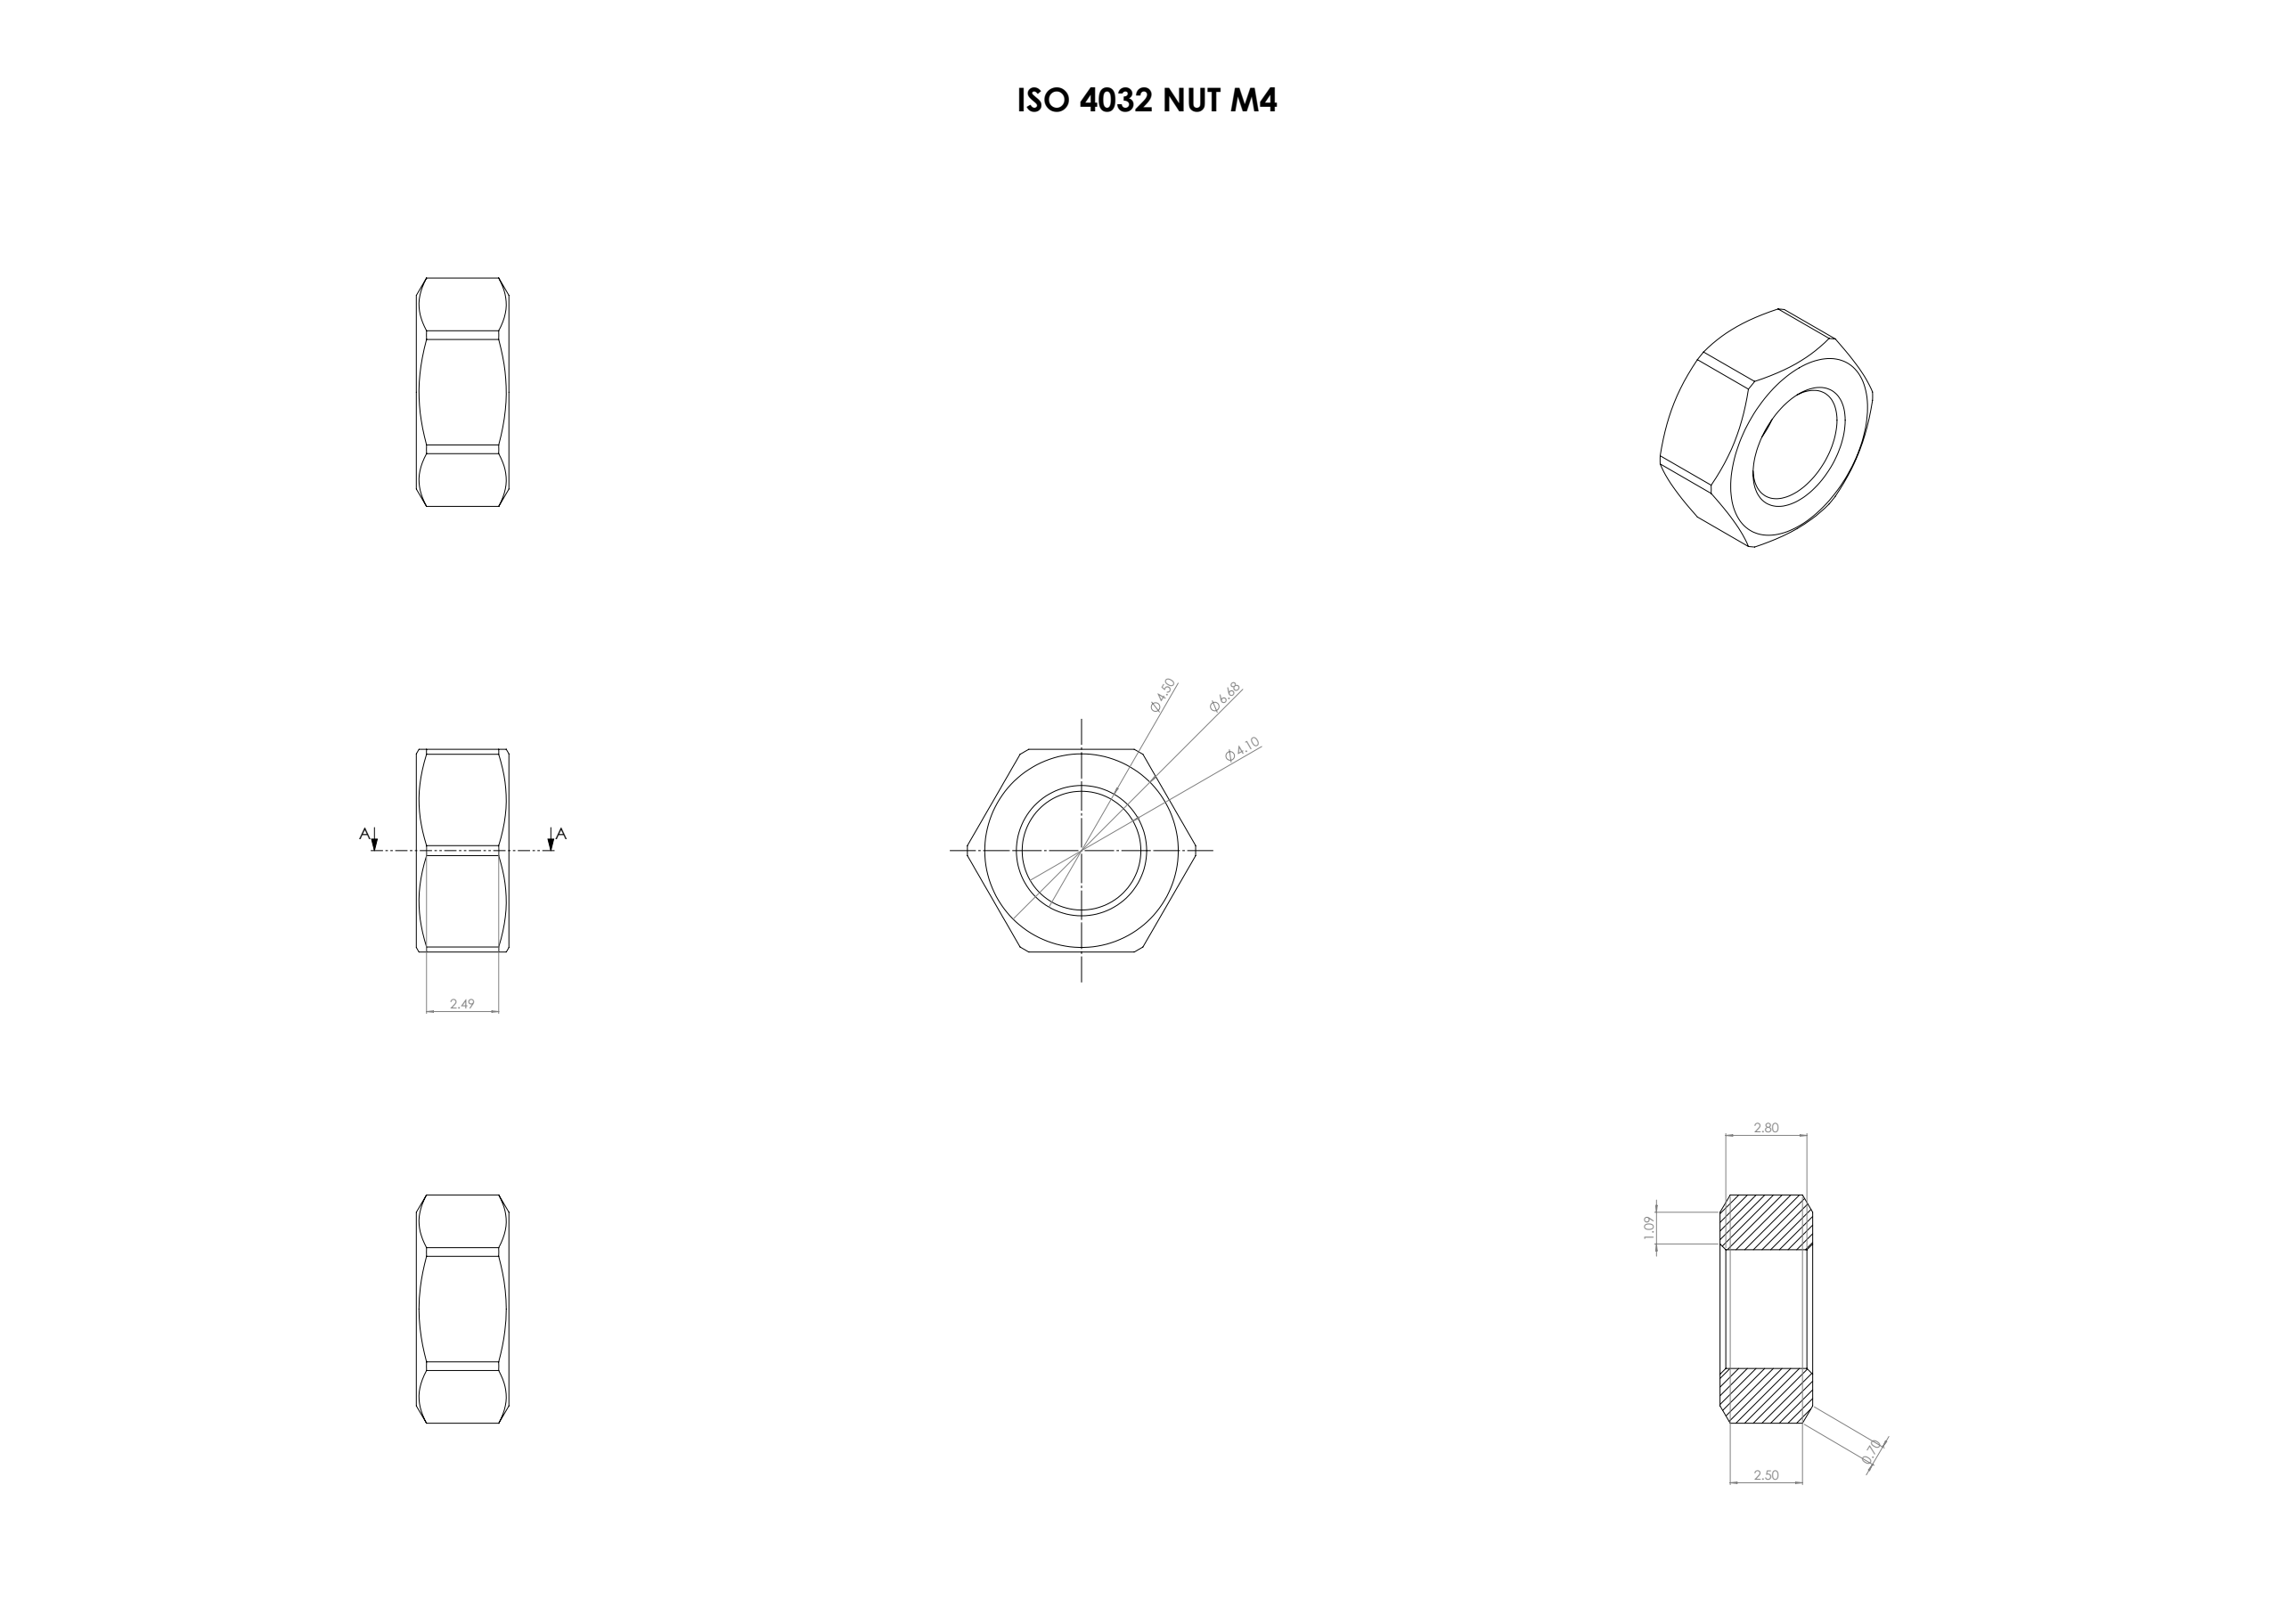
ISO-10303-21;
HEADER;
/* Generated by software containing ST-Developer
 * from STEP Tools, Inc. (www.steptools.com) 
 */

FILE_DESCRIPTION(
/* description */ (''),
/* implementation_level */ '2;1');

FILE_NAME(
/* name */ '10_ISO_4032_Nut_M4.step',
/* time_stamp */ '2026-10-21T02:01:14-07:00',
/* author */ (''),
/* organization */ (''),
/* preprocessor_version */ 'ST-DEVELOPER v20.2',
/* originating_system */ 'Autodesk Translation Framework v15.15.0.0',
/* authorisation */ '');

FILE_SCHEMA (('AUTOMOTIVE_DESIGN { 1 0 10303 214 3 1 1 }'));
ENDSEC;

DATA;
#10=MECHANICAL_DESIGN_GEOMETRIC_PRESENTATION_REPRESENTATION('',(#625),#37181);
#599=SHAPE_REPRESENTATION_RELATIONSHIP('SRR','None',#37249,#612);
#612=ADVANCED_BREP_SHAPE_REPRESENTATION('',(#638),#37179);
#625=STYLED_ITEM('',(#37380),#638);
#638=MANIFOLD_SOLID_BREP('Body1',#14787);
#686=FACE_BOUND('',#3028,.T.);
#687=FACE_BOUND('',#3031,.T.);
#912=CYLINDRICAL_SURFACE('',#16021,2.05);
#1265=CIRCLE('',#16017,3.34203030879952);
#1266=CIRCLE('',#16019,2.25);
#1267=CIRCLE('',#16020,2.05);
#1268=CIRCLE('',#16022,2.05);
#1269=CIRCLE('',#16024,3.34203030879952);
#1270=CIRCLE('',#16026,2.25);
#1362=CONICAL_SURFACE('',#16016,3.83322594216369,1.03985037524359);
#1363=CONICAL_SURFACE('',#16018,2.15,0.785398163397448);
#1364=CONICAL_SURFACE('',#16025,2.15,0.785398163397448);
#1365=CONICAL_SURFACE('',#16030,3.83322594216369,1.03985037524359);
#2136=FACE_OUTER_BOUND('',#3022,.T.);
#2137=FACE_OUTER_BOUND('',#3023,.T.);
#2138=FACE_OUTER_BOUND('',#3024,.T.);
#2139=FACE_OUTER_BOUND('',#3025,.T.);
#2140=FACE_OUTER_BOUND('',#3026,.T.);
#2141=FACE_OUTER_BOUND('',#3027,.T.);
#2142=FACE_OUTER_BOUND('',#3029,.T.);
#2143=FACE_OUTER_BOUND('',#3030,.T.);
#2144=FACE_OUTER_BOUND('',#3032,.T.);
#2145=FACE_OUTER_BOUND('',#3033,.T.);
#2146=FACE_OUTER_BOUND('',#3034,.T.);
#2147=FACE_OUTER_BOUND('',#3035,.T.);
#2148=FACE_OUTER_BOUND('',#3036,.T.);
#2149=FACE_OUTER_BOUND('',#3037,.T.);
#2150=FACE_OUTER_BOUND('',#3038,.T.);
#2151=FACE_OUTER_BOUND('',#3039,.T.);
#2152=FACE_OUTER_BOUND('',#3040,.T.);
#2153=FACE_OUTER_BOUND('',#3041,.T.);
#2154=FACE_OUTER_BOUND('',#3042,.T.);
#3022=EDGE_LOOP('',(#13069,#13070,#13071,#13072));
#3023=EDGE_LOOP('',(#13073,#13074,#13075,#13076));
#3024=EDGE_LOOP('',(#13077,#13078,#13079,#13080,#13081,#13082,#13083,#13084,
#13085,#13086,#13087,#13088,#13089,#13090,#13091,#13092));
#3025=EDGE_LOOP('',(#13093,#13094,#13095,#13096));
#3026=EDGE_LOOP('',(#13097,#13098,#13099,#13100));
#3027=EDGE_LOOP('',(#13101));
#3028=EDGE_LOOP('',(#13102));
#3029=EDGE_LOOP('',(#13103,#13104,#13105,#13106));
#3030=EDGE_LOOP('',(#13107));
#3031=EDGE_LOOP('',(#13108));
#3032=EDGE_LOOP('',(#13109,#13110,#13111,#13112));
#3033=EDGE_LOOP('',(#13113,#13114,#13115,#13116));
#3034=EDGE_LOOP('',(#13117,#13118,#13119,#13120,#13121,#13122,#13123,#13124,
#13125,#13126,#13127,#13128,#13129,#13130,#13131,#13132));
#3035=EDGE_LOOP('',(#13133,#13134,#13135,#13136));
#3036=EDGE_LOOP('',(#13137,#13138,#13139,#13140,#13141,#13142));
#3037=EDGE_LOOP('',(#13143,#13144,#13145,#13146));
#3038=EDGE_LOOP('',(#13147,#13148,#13149,#13150));
#3039=EDGE_LOOP('',(#13151,#13152,#13153,#13154));
#3040=EDGE_LOOP('',(#13155,#13156,#13157,#13158));
#3041=EDGE_LOOP('',(#13159,#13160,#13161,#13162));
#3042=EDGE_LOOP('',(#13163,#13164,#13165,#13166));
#3176=(
BOUNDED_CURVE()
B_SPLINE_CURVE(2,(#34308,#34309,#34310),.UNSPECIFIED.,.F.,.F.)
B_SPLINE_CURVE_WITH_KNOTS((3,3),(0.0719702485074244,0.107109429758004),
 .UNSPECIFIED.)
CURVE()
GEOMETRIC_REPRESENTATION_ITEM()
RATIONAL_B_SPLINE_CURVE((1.0121972483025,1.01317411304727,1.0121972483025))
REPRESENTATION_ITEM('')
);
#3177=(
BOUNDED_CURVE()
B_SPLINE_CURVE(2,(#34314,#34315,#34316),.UNSPECIFIED.,.F.,.F.)
B_SPLINE_CURVE_WITH_KNOTS((3,3),(0.0719702485074238,0.107109429758003),
 .UNSPECIFIED.)
CURVE()
GEOMETRIC_REPRESENTATION_ITEM()
RATIONAL_B_SPLINE_CURVE((1.0121972483025,1.01317411304726,1.0121972483025))
REPRESENTATION_ITEM('')
);
#3178=(
BOUNDED_CURVE()
B_SPLINE_CURVE(2,(#34320,#34321,#34322),.UNSPECIFIED.,.F.,.F.)
B_SPLINE_CURVE_WITH_KNOTS((3,3),(0.0663017168058462,0.456855245466122),
 .UNSPECIFIED.)
CURVE()
GEOMETRIC_REPRESENTATION_ITEM()
RATIONAL_B_SPLINE_CURVE((1.05321457643448,1.18720024765905,1.05321457643448))
REPRESENTATION_ITEM('')
);
#3179=(
BOUNDED_CURVE()
B_SPLINE_CURVE(2,(#34325,#34326,#34327),.UNSPECIFIED.,.F.,.F.)
B_SPLINE_CURVE_WITH_KNOTS((3,3),(0.0663017168058461,0.456855245466121),
 .UNSPECIFIED.)
CURVE()
GEOMETRIC_REPRESENTATION_ITEM()
RATIONAL_B_SPLINE_CURVE((1.05321457643448,1.18720024765905,1.05321457643448))
REPRESENTATION_ITEM('')
);
#3180=(
BOUNDED_CURVE()
B_SPLINE_CURVE(2,(#34330,#34331,#34332),.UNSPECIFIED.,.F.,.F.)
B_SPLINE_CURVE_WITH_KNOTS((3,3),(0.0663017168058462,0.456855245466121),
 .UNSPECIFIED.)
CURVE()
GEOMETRIC_REPRESENTATION_ITEM()
RATIONAL_B_SPLINE_CURVE((1.05321457643448,1.18720024765905,1.05321457643448))
REPRESENTATION_ITEM('')
);
#3181=(
BOUNDED_CURVE()
B_SPLINE_CURVE(2,(#34334,#34335,#34336),.UNSPECIFIED.,.F.,.F.)
B_SPLINE_CURVE_WITH_KNOTS((3,3),(0.0719702485074243,0.107109429758004),
 .UNSPECIFIED.)
CURVE()
GEOMETRIC_REPRESENTATION_ITEM()
RATIONAL_B_SPLINE_CURVE((1.0121972483025,1.01317411304726,1.0121972483025))
REPRESENTATION_ITEM('')
);
#3182=(
BOUNDED_CURVE()
B_SPLINE_CURVE(2,(#34338,#34339,#34340),.UNSPECIFIED.,.F.,.F.)
B_SPLINE_CURVE_WITH_KNOTS((3,3),(0.0663017168058464,0.456855245466122),
 .UNSPECIFIED.)
CURVE()
GEOMETRIC_REPRESENTATION_ITEM()
RATIONAL_B_SPLINE_CURVE((1.05321457643448,1.18720024765905,1.05321457643448))
REPRESENTATION_ITEM('')
);
#3183=(
BOUNDED_CURVE()
B_SPLINE_CURVE(2,(#34342,#34343,#34344),.UNSPECIFIED.,.F.,.F.)
B_SPLINE_CURVE_WITH_KNOTS((3,3),(0.0719702485074242,0.107109429758004),
 .UNSPECIFIED.)
CURVE()
GEOMETRIC_REPRESENTATION_ITEM()
RATIONAL_B_SPLINE_CURVE((1.0121972483025,1.01317411304726,1.0121972483025))
REPRESENTATION_ITEM('')
);
#3184=(
BOUNDED_CURVE()
B_SPLINE_CURVE(2,(#34346,#34347,#34348),.UNSPECIFIED.,.F.,.F.)
B_SPLINE_CURVE_WITH_KNOTS((3,3),(0.261578481135983,0.456855245466121),
 .UNSPECIFIED.)
CURVE()
GEOMETRIC_REPRESENTATION_ITEM()
RATIONAL_B_SPLINE_CURVE((1.12020741204677,1.12020741204677,1.05321457643449))
REPRESENTATION_ITEM('')
);
#3185=(
BOUNDED_CURVE()
B_SPLINE_CURVE(2,(#34353,#34354,#34355),.UNSPECIFIED.,.F.,.F.)
B_SPLINE_CURVE_WITH_KNOTS((3,3),(0.0663017168058461,0.261578481135983),
 .UNSPECIFIED.)
CURVE()
GEOMETRIC_REPRESENTATION_ITEM()
RATIONAL_B_SPLINE_CURVE((1.05321457643448,1.12020741204677,1.12020741204677))
REPRESENTATION_ITEM('')
);
#3186=(
BOUNDED_CURVE()
B_SPLINE_CURVE(2,(#34357,#34358,#34359),.UNSPECIFIED.,.F.,.F.)
B_SPLINE_CURVE_WITH_KNOTS((3,3),(0.0719702485074242,0.107109429758004),
 .UNSPECIFIED.)
CURVE()
GEOMETRIC_REPRESENTATION_ITEM()
RATIONAL_B_SPLINE_CURVE((1.0121972483025,1.01317411304727,1.0121972483025))
REPRESENTATION_ITEM('')
);
#3187=(
BOUNDED_CURVE()
B_SPLINE_CURVE(2,(#34361,#34362,#34363),.UNSPECIFIED.,.F.,.F.)
B_SPLINE_CURVE_WITH_KNOTS((3,3),(0.066301716805846,0.456855245466121),
 .UNSPECIFIED.)
CURVE()
GEOMETRIC_REPRESENTATION_ITEM()
RATIONAL_B_SPLINE_CURVE((1.05321457643448,1.18720024765905,1.05321457643448))
REPRESENTATION_ITEM('')
);
#3188=(
BOUNDED_CURVE()
B_SPLINE_CURVE(2,(#34365,#34366,#34367),.UNSPECIFIED.,.F.,.F.)
B_SPLINE_CURVE_WITH_KNOTS((3,3),(0.0719702485074249,0.107109429758004),
 .UNSPECIFIED.)
CURVE()
GEOMETRIC_REPRESENTATION_ITEM()
RATIONAL_B_SPLINE_CURVE((1.0121972483025,1.01317411304726,1.0121972483025))
REPRESENTATION_ITEM('')
);
#3189=(
BOUNDED_CURVE()
B_SPLINE_CURVE(2,(#34369,#34370,#34371),.UNSPECIFIED.,.F.,.F.)
B_SPLINE_CURVE_WITH_KNOTS((3,3),(0.0663017168058463,0.456855245466121),
 .UNSPECIFIED.)
CURVE()
GEOMETRIC_REPRESENTATION_ITEM()
RATIONAL_B_SPLINE_CURVE((1.05321457643448,1.18720024765905,1.05321457643448))
REPRESENTATION_ITEM('')
);
#3190=(
BOUNDED_CURVE()
B_SPLINE_CURVE(2,(#34372,#34373,#34374),.UNSPECIFIED.,.F.,.F.)
B_SPLINE_CURVE_WITH_KNOTS((3,3),(0.0719702485074235,0.107109429758003),
 .UNSPECIFIED.)
CURVE()
GEOMETRIC_REPRESENTATION_ITEM()
RATIONAL_B_SPLINE_CURVE((1.0121972483025,1.01317411304727,1.0121972483025))
REPRESENTATION_ITEM('')
);
#3191=(
BOUNDED_CURVE()
B_SPLINE_CURVE(2,(#34397,#34398,#34399),.UNSPECIFIED.,.F.,.F.)
B_SPLINE_CURVE_WITH_KNOTS((3,3),(0.0719702485074245,0.107109429758004),
 .UNSPECIFIED.)
CURVE()
GEOMETRIC_REPRESENTATION_ITEM()
RATIONAL_B_SPLINE_CURVE((1.0121972483025,1.01317411304727,1.0121972483025))
REPRESENTATION_ITEM('')
);
#3192=(
BOUNDED_CURVE()
B_SPLINE_CURVE(2,(#34403,#34404,#34405),.UNSPECIFIED.,.F.,.F.)
B_SPLINE_CURVE_WITH_KNOTS((3,3),(0.0663017168058461,0.456855245466121),
 .UNSPECIFIED.)
CURVE()
GEOMETRIC_REPRESENTATION_ITEM()
RATIONAL_B_SPLINE_CURVE((1.05321457643448,1.18720024765905,1.05321457643448))
REPRESENTATION_ITEM('')
);
#3193=(
BOUNDED_CURVE()
B_SPLINE_CURVE(2,(#34411,#34412,#34413),.UNSPECIFIED.,.F.,.F.)
B_SPLINE_CURVE_WITH_KNOTS((3,3),(0.0663017168058461,0.261578481135983),
 .UNSPECIFIED.)
CURVE()
GEOMETRIC_REPRESENTATION_ITEM()
RATIONAL_B_SPLINE_CURVE((1.05321457643448,1.12020741204677,1.12020741204677))
REPRESENTATION_ITEM('')
);
#3194=(
BOUNDED_CURVE()
B_SPLINE_CURVE(2,(#34414,#34415,#34416),.UNSPECIFIED.,.F.,.F.)
B_SPLINE_CURVE_WITH_KNOTS((3,3),(0.0719702485074254,0.107109429758005),
 .UNSPECIFIED.)
CURVE()
GEOMETRIC_REPRESENTATION_ITEM()
RATIONAL_B_SPLINE_CURVE((1.0121972483025,1.01317411304726,1.0121972483025))
REPRESENTATION_ITEM('')
);
#3195=(
BOUNDED_CURVE()
B_SPLINE_CURVE(2,(#34417,#34418,#34419),.UNSPECIFIED.,.F.,.F.)
B_SPLINE_CURVE_WITH_KNOTS((3,3),(0.0663017168058463,0.456855245466121),
 .UNSPECIFIED.)
CURVE()
GEOMETRIC_REPRESENTATION_ITEM()
RATIONAL_B_SPLINE_CURVE((1.05321457643448,1.18720024765905,1.05321457643448))
REPRESENTATION_ITEM('')
);
#3196=(
BOUNDED_CURVE()
B_SPLINE_CURVE(2,(#34421,#34422,#34423),.UNSPECIFIED.,.F.,.F.)
B_SPLINE_CURVE_WITH_KNOTS((3,3),(0.0719702485074251,0.107109429758005),
 .UNSPECIFIED.)
CURVE()
GEOMETRIC_REPRESENTATION_ITEM()
RATIONAL_B_SPLINE_CURVE((1.0121972483025,1.01317411304726,1.01219724830249))
REPRESENTATION_ITEM('')
);
#3197=(
BOUNDED_CURVE()
B_SPLINE_CURVE(2,(#34425,#34426,#34427),.UNSPECIFIED.,.F.,.F.)
B_SPLINE_CURVE_WITH_KNOTS((3,3),(0.0663017168058462,0.456855245466121),
 .UNSPECIFIED.)
CURVE()
GEOMETRIC_REPRESENTATION_ITEM()
RATIONAL_B_SPLINE_CURVE((1.05321457643448,1.18720024765905,1.05321457643448))
REPRESENTATION_ITEM('')
);
#3198=(
BOUNDED_CURVE()
B_SPLINE_CURVE(2,(#34429,#34430,#34431),.UNSPECIFIED.,.F.,.F.)
B_SPLINE_CURVE_WITH_KNOTS((3,3),(0.0719702485074238,0.107109429758004),
 .UNSPECIFIED.)
CURVE()
GEOMETRIC_REPRESENTATION_ITEM()
RATIONAL_B_SPLINE_CURVE((1.0121972483025,1.01317411304727,1.0121972483025))
REPRESENTATION_ITEM('')
);
#3199=(
BOUNDED_CURVE()
B_SPLINE_CURVE(2,(#34433,#34434,#34435),.UNSPECIFIED.,.F.,.F.)
B_SPLINE_CURVE_WITH_KNOTS((3,3),(0.0663017168058462,0.456855245466121),
 .UNSPECIFIED.)
CURVE()
GEOMETRIC_REPRESENTATION_ITEM()
RATIONAL_B_SPLINE_CURVE((1.05321457643448,1.18720024765905,1.05321457643448))
REPRESENTATION_ITEM('')
);
#3200=(
BOUNDED_CURVE()
B_SPLINE_CURVE(2,(#34437,#34438,#34439),.UNSPECIFIED.,.F.,.F.)
B_SPLINE_CURVE_WITH_KNOTS((3,3),(0.0719702485074251,0.107109429758005),
 .UNSPECIFIED.)
CURVE()
GEOMETRIC_REPRESENTATION_ITEM()
RATIONAL_B_SPLINE_CURVE((1.0121972483025,1.01317411304726,1.0121972483025))
REPRESENTATION_ITEM('')
);
#3201=(
BOUNDED_CURVE()
B_SPLINE_CURVE(2,(#34440,#34441,#34442),.UNSPECIFIED.,.F.,.F.)
B_SPLINE_CURVE_WITH_KNOTS((3,3),(0.261578481135983,0.456855245466121),
 .UNSPECIFIED.)
CURVE()
GEOMETRIC_REPRESENTATION_ITEM()
RATIONAL_B_SPLINE_CURVE((1.12020741204677,1.12020741204677,1.05321457643448))
REPRESENTATION_ITEM('')
);
#4375=LINE('',#34312,#5614);
#4376=LINE('',#34317,#5615);
#4377=LINE('',#34324,#5616);
#4378=LINE('',#34350,#5617);
#4379=LINE('',#34379,#5618);
#4380=LINE('',#34383,#5619);
#4381=LINE('',#34391,#5620);
#4382=LINE('',#34395,#5621);
#4383=LINE('',#34400,#5622);
#4384=LINE('',#34406,#5623);
#4385=LINE('',#34409,#5624);
#4386=LINE('',#34444,#5625);
#4387=LINE('',#34446,#5626);
#4388=LINE('',#34448,#5627);
#4389=LINE('',#34450,#5628);
#4390=LINE('',#34452,#5629);
#4391=LINE('',#34454,#5630);
#5614=VECTOR('',#19461,10.);
#5615=VECTOR('',#19462,10.);
#5616=VECTOR('',#19465,10.);
#5617=VECTOR('',#19468,3.83322594216369);
#5618=VECTOR('',#19475,2.15);
#5619=VECTOR('',#19480,2.05);
#5620=VECTOR('',#19491,2.15);
#5621=VECTOR('',#19496,10.);
#5622=VECTOR('',#19497,10.);
#5623=VECTOR('',#19500,10.);
#5624=VECTOR('',#19503,3.83322594216369);
#5625=VECTOR('',#19506,10.);
#5626=VECTOR('',#19509,10.);
#5627=VECTOR('',#19512,10.);
#5628=VECTOR('',#19515,10.);
#5629=VECTOR('',#19518,10.);
#5630=VECTOR('',#19521,10.);
#6898=VERTEX_POINT('',#34306);
#6899=VERTEX_POINT('',#34307);
#6900=VERTEX_POINT('',#34311);
#6901=VERTEX_POINT('',#34313);
#6902=VERTEX_POINT('',#34319);
#6903=VERTEX_POINT('',#34323);
#6904=VERTEX_POINT('',#34329);
#6905=VERTEX_POINT('',#34333);
#6906=VERTEX_POINT('',#34337);
#6907=VERTEX_POINT('',#34341);
#6908=VERTEX_POINT('',#34345);
#6909=VERTEX_POINT('',#34349);
#6910=VERTEX_POINT('',#34352);
#6911=VERTEX_POINT('',#34356);
#6912=VERTEX_POINT('',#34360);
#6913=VERTEX_POINT('',#34364);
#6914=VERTEX_POINT('',#34368);
#6915=VERTEX_POINT('',#34376);
#6916=VERTEX_POINT('',#34378);
#6917=VERTEX_POINT('',#34382);
#6918=VERTEX_POINT('',#34386);
#6919=VERTEX_POINT('',#34389);
#6920=VERTEX_POINT('',#34394);
#6921=VERTEX_POINT('',#34396);
#6922=VERTEX_POINT('',#34402);
#6923=VERTEX_POINT('',#34408);
#6924=VERTEX_POINT('',#34410);
#6925=VERTEX_POINT('',#34420);
#6926=VERTEX_POINT('',#34424);
#6927=VERTEX_POINT('',#34428);
#6928=VERTEX_POINT('',#34432);
#6929=VERTEX_POINT('',#34436);
#8976=EDGE_CURVE('',#6898,#6899,#3176,.T.);
#8977=EDGE_CURVE('',#6899,#6900,#4375,.T.);
#8978=EDGE_CURVE('',#6900,#6901,#3177,.T.);
#8979=EDGE_CURVE('',#6901,#6898,#4376,.T.);
#8980=EDGE_CURVE('',#6899,#6902,#3178,.T.);
#8981=EDGE_CURVE('',#6903,#6902,#4377,.T.);
#8982=EDGE_CURVE('',#6903,#6900,#3179,.T.);
#8983=EDGE_CURVE('',#6904,#6898,#3180,.T.);
#8984=EDGE_CURVE('',#6905,#6904,#3181,.T.);
#8985=EDGE_CURVE('',#6906,#6905,#3182,.T.);
#8986=EDGE_CURVE('',#6907,#6906,#3183,.T.);
#8987=EDGE_CURVE('',#6908,#6907,#3184,.T.);
#8988=EDGE_CURVE('',#6908,#6909,#4378,.T.);
#8989=EDGE_CURVE('',#6909,#6909,#1265,.T.);
#8990=EDGE_CURVE('',#6910,#6908,#3185,.T.);
#8991=EDGE_CURVE('',#6911,#6910,#3186,.T.);
#8992=EDGE_CURVE('',#6912,#6911,#3187,.T.);
#8993=EDGE_CURVE('',#6913,#6912,#3188,.T.);
#8994=EDGE_CURVE('',#6914,#6913,#3189,.T.);
#8995=EDGE_CURVE('',#6902,#6914,#3190,.T.);
#8996=EDGE_CURVE('',#6915,#6915,#1266,.T.);
#8997=EDGE_CURVE('',#6915,#6916,#4379,.T.);
#8998=EDGE_CURVE('',#6916,#6916,#1267,.T.);
#8999=EDGE_CURVE('',#6916,#6917,#4380,.T.);
#9000=EDGE_CURVE('',#6917,#6917,#1268,.T.);
#9001=EDGE_CURVE('',#6918,#6918,#1269,.T.);
#9002=EDGE_CURVE('',#6919,#6919,#1270,.T.);
#9003=EDGE_CURVE('',#6919,#6917,#4381,.T.);
#9004=EDGE_CURVE('',#6904,#6920,#4382,.T.);
#9005=EDGE_CURVE('',#6920,#6921,#3191,.T.);
#9006=EDGE_CURVE('',#6921,#6905,#4383,.T.);
#9007=EDGE_CURVE('',#6921,#6922,#3192,.T.);
#9008=EDGE_CURVE('',#6906,#6922,#4384,.T.);
#9009=EDGE_CURVE('',#6918,#6923,#4385,.T.);
#9010=EDGE_CURVE('',#6924,#6923,#3193,.T.);
#9011=EDGE_CURVE('',#6922,#6924,#3194,.T.);
#9012=EDGE_CURVE('',#6901,#6920,#3195,.T.);
#9013=EDGE_CURVE('',#6925,#6903,#3196,.T.);
#9014=EDGE_CURVE('',#6926,#6925,#3197,.T.);
#9015=EDGE_CURVE('',#6927,#6926,#3198,.T.);
#9016=EDGE_CURVE('',#6928,#6927,#3199,.T.);
#9017=EDGE_CURVE('',#6929,#6928,#3200,.T.);
#9018=EDGE_CURVE('',#6923,#6929,#3201,.T.);
#9019=EDGE_CURVE('',#6924,#6907,#4386,.T.);
#9020=EDGE_CURVE('',#6910,#6929,#4387,.T.);
#9021=EDGE_CURVE('',#6928,#6911,#4388,.T.);
#9022=EDGE_CURVE('',#6914,#6925,#4389,.T.);
#9023=EDGE_CURVE('',#6926,#6913,#4390,.T.);
#9024=EDGE_CURVE('',#6912,#6927,#4391,.T.);
#13069=ORIENTED_EDGE('',*,*,#8976,.T.);
#13070=ORIENTED_EDGE('',*,*,#8977,.T.);
#13071=ORIENTED_EDGE('',*,*,#8978,.T.);
#13072=ORIENTED_EDGE('',*,*,#8979,.T.);
#13073=ORIENTED_EDGE('',*,*,#8977,.F.);
#13074=ORIENTED_EDGE('',*,*,#8980,.T.);
#13075=ORIENTED_EDGE('',*,*,#8981,.F.);
#13076=ORIENTED_EDGE('',*,*,#8982,.T.);
#13077=ORIENTED_EDGE('',*,*,#8976,.F.);
#13078=ORIENTED_EDGE('',*,*,#8983,.F.);
#13079=ORIENTED_EDGE('',*,*,#8984,.F.);
#13080=ORIENTED_EDGE('',*,*,#8985,.F.);
#13081=ORIENTED_EDGE('',*,*,#8986,.F.);
#13082=ORIENTED_EDGE('',*,*,#8987,.F.);
#13083=ORIENTED_EDGE('',*,*,#8988,.T.);
#13084=ORIENTED_EDGE('',*,*,#8989,.F.);
#13085=ORIENTED_EDGE('',*,*,#8988,.F.);
#13086=ORIENTED_EDGE('',*,*,#8990,.F.);
#13087=ORIENTED_EDGE('',*,*,#8991,.F.);
#13088=ORIENTED_EDGE('',*,*,#8992,.F.);
#13089=ORIENTED_EDGE('',*,*,#8993,.F.);
#13090=ORIENTED_EDGE('',*,*,#8994,.F.);
#13091=ORIENTED_EDGE('',*,*,#8995,.F.);
#13092=ORIENTED_EDGE('',*,*,#8980,.F.);
#13093=ORIENTED_EDGE('',*,*,#8996,.T.);
#13094=ORIENTED_EDGE('',*,*,#8997,.T.);
#13095=ORIENTED_EDGE('',*,*,#8998,.T.);
#13096=ORIENTED_EDGE('',*,*,#8997,.F.);
#13097=ORIENTED_EDGE('',*,*,#8998,.F.);
#13098=ORIENTED_EDGE('',*,*,#8999,.T.);
#13099=ORIENTED_EDGE('',*,*,#9000,.F.);
#13100=ORIENTED_EDGE('',*,*,#8999,.F.);
#13101=ORIENTED_EDGE('',*,*,#9001,.T.);
#13102=ORIENTED_EDGE('',*,*,#8996,.F.);
#13103=ORIENTED_EDGE('',*,*,#9002,.T.);
#13104=ORIENTED_EDGE('',*,*,#9003,.T.);
#13105=ORIENTED_EDGE('',*,*,#9000,.T.);
#13106=ORIENTED_EDGE('',*,*,#9003,.F.);
#13107=ORIENTED_EDGE('',*,*,#8989,.T.);
#13108=ORIENTED_EDGE('',*,*,#9002,.F.);
#13109=ORIENTED_EDGE('',*,*,#8984,.T.);
#13110=ORIENTED_EDGE('',*,*,#9004,.T.);
#13111=ORIENTED_EDGE('',*,*,#9005,.T.);
#13112=ORIENTED_EDGE('',*,*,#9006,.T.);
#13113=ORIENTED_EDGE('',*,*,#9006,.F.);
#13114=ORIENTED_EDGE('',*,*,#9007,.T.);
#13115=ORIENTED_EDGE('',*,*,#9008,.F.);
#13116=ORIENTED_EDGE('',*,*,#8985,.T.);
#13117=ORIENTED_EDGE('',*,*,#9001,.F.);
#13118=ORIENTED_EDGE('',*,*,#9009,.T.);
#13119=ORIENTED_EDGE('',*,*,#9010,.F.);
#13120=ORIENTED_EDGE('',*,*,#9011,.F.);
#13121=ORIENTED_EDGE('',*,*,#9007,.F.);
#13122=ORIENTED_EDGE('',*,*,#9005,.F.);
#13123=ORIENTED_EDGE('',*,*,#9012,.F.);
#13124=ORIENTED_EDGE('',*,*,#8978,.F.);
#13125=ORIENTED_EDGE('',*,*,#8982,.F.);
#13126=ORIENTED_EDGE('',*,*,#9013,.F.);
#13127=ORIENTED_EDGE('',*,*,#9014,.F.);
#13128=ORIENTED_EDGE('',*,*,#9015,.F.);
#13129=ORIENTED_EDGE('',*,*,#9016,.F.);
#13130=ORIENTED_EDGE('',*,*,#9017,.F.);
#13131=ORIENTED_EDGE('',*,*,#9018,.F.);
#13132=ORIENTED_EDGE('',*,*,#9009,.F.);
#13133=ORIENTED_EDGE('',*,*,#8986,.T.);
#13134=ORIENTED_EDGE('',*,*,#9008,.T.);
#13135=ORIENTED_EDGE('',*,*,#9011,.T.);
#13136=ORIENTED_EDGE('',*,*,#9019,.T.);
#13137=ORIENTED_EDGE('',*,*,#9019,.F.);
#13138=ORIENTED_EDGE('',*,*,#9010,.T.);
#13139=ORIENTED_EDGE('',*,*,#9018,.T.);
#13140=ORIENTED_EDGE('',*,*,#9020,.F.);
#13141=ORIENTED_EDGE('',*,*,#8990,.T.);
#13142=ORIENTED_EDGE('',*,*,#8987,.T.);
#13143=ORIENTED_EDGE('',*,*,#8991,.T.);
#13144=ORIENTED_EDGE('',*,*,#9020,.T.);
#13145=ORIENTED_EDGE('',*,*,#9017,.T.);
#13146=ORIENTED_EDGE('',*,*,#9021,.T.);
#13147=ORIENTED_EDGE('',*,*,#8995,.T.);
#13148=ORIENTED_EDGE('',*,*,#9022,.T.);
#13149=ORIENTED_EDGE('',*,*,#9013,.T.);
#13150=ORIENTED_EDGE('',*,*,#8981,.T.);
#13151=ORIENTED_EDGE('',*,*,#9022,.F.);
#13152=ORIENTED_EDGE('',*,*,#8994,.T.);
#13153=ORIENTED_EDGE('',*,*,#9023,.F.);
#13154=ORIENTED_EDGE('',*,*,#9014,.T.);
#13155=ORIENTED_EDGE('',*,*,#8993,.T.);
#13156=ORIENTED_EDGE('',*,*,#9024,.T.);
#13157=ORIENTED_EDGE('',*,*,#9015,.T.);
#13158=ORIENTED_EDGE('',*,*,#9023,.T.);
#13159=ORIENTED_EDGE('',*,*,#9021,.F.);
#13160=ORIENTED_EDGE('',*,*,#9016,.T.);
#13161=ORIENTED_EDGE('',*,*,#9024,.F.);
#13162=ORIENTED_EDGE('',*,*,#8992,.T.);
#13163=ORIENTED_EDGE('',*,*,#8979,.F.);
#13164=ORIENTED_EDGE('',*,*,#9012,.T.);
#13165=ORIENTED_EDGE('',*,*,#9004,.F.);
#13166=ORIENTED_EDGE('',*,*,#8983,.T.);
#13912=PLANE('',#16014);
#13913=PLANE('',#16015);
#13914=PLANE('',#16023);
#13915=PLANE('',#16027);
#13916=PLANE('',#16028);
#13917=PLANE('',#16029);
#13918=PLANE('',#16031);
#13919=PLANE('',#16032);
#13920=PLANE('',#16033);
#13921=PLANE('',#16034);
#13922=PLANE('',#16035);
#13923=PLANE('',#16036);
#13924=PLANE('',#16037);
#13925=PLANE('',#16038);
#14704=ADVANCED_FACE('',(#2136),#13912,.T.);
#14705=ADVANCED_FACE('',(#2137),#13913,.T.);
#14706=ADVANCED_FACE('',(#2138),#1362,.T.);
#14707=ADVANCED_FACE('',(#2139),#1363,.F.);
#14708=ADVANCED_FACE('',(#2140),#912,.F.);
#14709=ADVANCED_FACE('',(#2141,#686),#13914,.F.);
#14710=ADVANCED_FACE('',(#2142),#1364,.F.);
#14711=ADVANCED_FACE('',(#2143,#687),#13915,.T.);
#14712=ADVANCED_FACE('',(#2144),#13916,.T.);
#14713=ADVANCED_FACE('',(#2145),#13917,.T.);
#14714=ADVANCED_FACE('',(#2146),#1365,.T.);
#14715=ADVANCED_FACE('',(#2147),#13918,.T.);
#14716=ADVANCED_FACE('',(#2148),#13919,.T.);
#14717=ADVANCED_FACE('',(#2149),#13920,.T.);
#14718=ADVANCED_FACE('',(#2150),#13921,.T.);
#14719=ADVANCED_FACE('',(#2151),#13922,.T.);
#14720=ADVANCED_FACE('',(#2152),#13923,.T.);
#14721=ADVANCED_FACE('',(#2153),#13924,.T.);
#14722=ADVANCED_FACE('',(#2154),#13925,.T.);
#14787=CLOSED_SHELL('',(#14704,#14705,#14706,#14707,#14708,#14709,#14710,
#14711,#14712,#14713,#14714,#14715,#14716,#14717,#14718,#14719,#14720,#14721,
#14722));
#16013=AXIS2_PLACEMENT_3D('',#34304,#19457,#19458);
#16014=AXIS2_PLACEMENT_3D('',#34305,#19459,#19460);
#16015=AXIS2_PLACEMENT_3D('',#34318,#19463,#19464);
#16016=AXIS2_PLACEMENT_3D('',#34328,#19466,#19467);
#16017=AXIS2_PLACEMENT_3D('',#34351,#19469,#19470);
#16018=AXIS2_PLACEMENT_3D('',#34375,#19471,#19472);
#16019=AXIS2_PLACEMENT_3D('',#34377,#19473,#19474);
#16020=AXIS2_PLACEMENT_3D('',#34380,#19476,#19477);
#16021=AXIS2_PLACEMENT_3D('',#34381,#19478,#19479);
#16022=AXIS2_PLACEMENT_3D('',#34384,#19481,#19482);
#16023=AXIS2_PLACEMENT_3D('',#34385,#19483,#19484);
#16024=AXIS2_PLACEMENT_3D('',#34387,#19485,#19486);
#16025=AXIS2_PLACEMENT_3D('',#34388,#19487,#19488);
#16026=AXIS2_PLACEMENT_3D('',#34390,#19489,#19490);
#16027=AXIS2_PLACEMENT_3D('',#34392,#19492,#19493);
#16028=AXIS2_PLACEMENT_3D('',#34393,#19494,#19495);
#16029=AXIS2_PLACEMENT_3D('',#34401,#19498,#19499);
#16030=AXIS2_PLACEMENT_3D('',#34407,#19501,#19502);
#16031=AXIS2_PLACEMENT_3D('',#34443,#19504,#19505);
#16032=AXIS2_PLACEMENT_3D('',#34445,#19507,#19508);
#16033=AXIS2_PLACEMENT_3D('',#34447,#19510,#19511);
#16034=AXIS2_PLACEMENT_3D('',#34449,#19513,#19514);
#16035=AXIS2_PLACEMENT_3D('',#34451,#19516,#19517);
#16036=AXIS2_PLACEMENT_3D('',#34453,#19519,#19520);
#16037=AXIS2_PLACEMENT_3D('',#34455,#19522,#19523);
#16038=AXIS2_PLACEMENT_3D('',#34456,#19524,#19525);
#19457=DIRECTION('axis',(0.,0.,1.));
#19458=DIRECTION('refdir',(1.,0.,0.));
#19459=DIRECTION('center_axis',(0.,0.866025403784439,0.5));
#19460=DIRECTION('ref_axis',(1.,0.,0.));
#19461=DIRECTION('',(-1.,0.,0.));
#19462=DIRECTION('',(1.,0.,0.));
#19463=DIRECTION('center_axis',(0.,1.,-2.74708955197652E-16));
#19464=DIRECTION('ref_axis',(0.,2.74708955197652E-16,1.));
#19465=DIRECTION('',(1.,0.,0.));
#19466=DIRECTION('center_axis',(-1.,0.,0.));
#19467=DIRECTION('ref_axis',(0.,1.,0.));
#19468=DIRECTION('',(0.506349288588207,0.862328474507375,1.05604780611908E-16));
#19469=DIRECTION('center_axis',(1.,0.,0.));
#19470=DIRECTION('ref_axis',(0.,1.,0.));
#19471=DIRECTION('center_axis',(-1.,0.,0.));
#19472=DIRECTION('ref_axis',(0.,0.,-1.));
#19473=DIRECTION('center_axis',(-1.,0.,0.));
#19474=DIRECTION('ref_axis',(0.,0.,-1.));
#19475=DIRECTION('',(0.707106781186548,-8.65956056235493E-17,-0.707106781186547));
#19476=DIRECTION('center_axis',(1.,0.,0.));
#19477=DIRECTION('ref_axis',(0.,0.,-1.));
#19478=DIRECTION('center_axis',(1.,0.,0.));
#19479=DIRECTION('ref_axis',(0.,0.,-1.));
#19480=DIRECTION('',(1.,0.,0.));
#19481=DIRECTION('center_axis',(-1.,0.,0.));
#19482=DIRECTION('ref_axis',(0.,0.,-1.));
#19483=DIRECTION('center_axis',(1.,0.,0.));
#19484=DIRECTION('ref_axis',(0.,0.,-1.));
#19485=DIRECTION('center_axis',(-1.,0.,0.));
#19486=DIRECTION('ref_axis',(0.,1.,0.));
#19487=DIRECTION('center_axis',(1.,0.,0.));
#19488=DIRECTION('ref_axis',(0.,0.,-1.));
#19489=DIRECTION('center_axis',(1.,0.,0.));
#19490=DIRECTION('ref_axis',(0.,0.,-1.));
#19491=DIRECTION('',(-0.707106781186548,8.65956056235493E-17,-0.707106781186547));
#19492=DIRECTION('center_axis',(1.,0.,0.));
#19493=DIRECTION('ref_axis',(0.,0.,-1.));
#19494=DIRECTION('center_axis',(0.,0.,1.));
#19495=DIRECTION('ref_axis',(1.,0.,0.));
#19496=DIRECTION('',(-1.,0.,0.));
#19497=DIRECTION('',(1.,0.,0.));
#19498=DIRECTION('center_axis',(0.,-0.5,0.866025403784439));
#19499=DIRECTION('ref_axis',(0.,-0.866025403784439,-0.5));
#19500=DIRECTION('',(-1.,0.,0.));
#19501=DIRECTION('center_axis',(1.,0.,0.));
#19502=DIRECTION('ref_axis',(0.,1.,0.));
#19503=DIRECTION('',(0.506349288588206,-0.862328474507375,-1.05604780611908E-16));
#19504=DIRECTION('center_axis',(0.,-0.866025403784438,0.500000000000002));
#19505=DIRECTION('ref_axis',(1.,0.,0.));
#19506=DIRECTION('',(1.,0.,0.));
#19507=DIRECTION('center_axis',(0.,-1.,-1.37354477598826E-16));
#19508=DIRECTION('ref_axis',(0.,1.37354477598826E-16,-1.));
#19509=DIRECTION('',(-1.,0.,0.));
#19510=DIRECTION('center_axis',(0.,-0.866025403784439,-0.499999999999999));
#19511=DIRECTION('ref_axis',(0.,0.499999999999999,-0.866025403784439));
#19512=DIRECTION('',(1.,0.,0.));
#19513=DIRECTION('center_axis',(0.,0.866025403784438,-0.500000000000002));
#19514=DIRECTION('ref_axis',(-1.,0.,0.));
#19515=DIRECTION('',(-1.,0.,0.));
#19516=DIRECTION('center_axis',(0.,0.5,-0.866025403784439));
#19517=DIRECTION('ref_axis',(0.,0.866025403784439,0.5));
#19518=DIRECTION('',(1.,0.,0.));
#19519=DIRECTION('center_axis',(0.,1.60246890531963E-15,-1.));
#19520=DIRECTION('ref_axis',(-1.,0.,0.));
#19521=DIRECTION('',(-1.,0.,0.));
#19522=DIRECTION('center_axis',(0.,-0.5,-0.866025403784439));
#19523=DIRECTION('ref_axis',(0.,0.866025403784439,-0.5));
#19524=DIRECTION('center_axis',(0.,0.5,0.866025403784439));
#19525=DIRECTION('ref_axis',(0.,-0.866025403784439,0.5));
#34304=CARTESIAN_POINT('',(0.,0.,0.));
#34305=CARTESIAN_POINT('Origin',(0.,3.41339745962156,1.97072594216369));
#34306=CARTESIAN_POINT('',(2.84579300863683,3.32679491924311,2.12072594216369));
#34307=CARTESIAN_POINT('',(2.84579300863683,3.5,1.82072594216369));
#34308=CARTESIAN_POINT('Ctrl Pts',(2.84579300863683,3.32679491924311,2.12072594216369));
#34309=CARTESIAN_POINT('Ctrl Pts',(2.85025803029788,3.41339745962156,1.97072594216368));
#34310=CARTESIAN_POINT('Ctrl Pts',(2.84579300863683,3.5,1.82072594216369));
#34311=CARTESIAN_POINT('',(0.35420699136317,3.5,1.82072594216369));
#34312=CARTESIAN_POINT('',(0.,3.5,1.82072594216369));
#34313=CARTESIAN_POINT('',(0.35420699136317,3.32679491924311,2.12072594216369));
#34314=CARTESIAN_POINT('Ctrl Pts',(0.35420699136317,3.5,1.82072594216369));
#34315=CARTESIAN_POINT('Ctrl Pts',(0.349741969702116,3.41339745962155,1.9707259421637));
#34316=CARTESIAN_POINT('Ctrl Pts',(0.35420699136317,3.32679491924311,2.12072594216369));
#34317=CARTESIAN_POINT('',(0.,3.32679491924311,2.12072594216369));
#34318=CARTESIAN_POINT('Origin',(0.,3.5,-2.02072594216369));
#34319=CARTESIAN_POINT('',(2.84579300863683,3.5,-1.82072594216369));
#34320=CARTESIAN_POINT('Ctrl Pts',(2.84579300863683,3.5,1.82072594216369));
#34321=CARTESIAN_POINT('Ctrl Pts',(3.3391842955686,3.5,-3.60822483003176E-15));
#34322=CARTESIAN_POINT('Ctrl Pts',(2.84579300863683,3.5,-1.82072594216369));
#34323=CARTESIAN_POINT('',(0.35420699136317,3.5,-1.82072594216369));
#34324=CARTESIAN_POINT('',(0.,3.5,-1.82072594216369));
#34325=CARTESIAN_POINT('Ctrl Pts',(0.35420699136317,3.5,-1.82072594216369));
#34326=CARTESIAN_POINT('Ctrl Pts',(-0.139184295568601,3.5,3.05311331771918E-15));
#34327=CARTESIAN_POINT('Ctrl Pts',(0.35420699136317,3.5,1.82072594216369));
#34328=CARTESIAN_POINT('Origin',(2.91157561548264,0.,0.));
#34329=CARTESIAN_POINT('',(2.84579300863683,0.173205080756888,3.94145188432738));
#34330=CARTESIAN_POINT('Ctrl Pts',(2.84579300863683,0.173205080756888,3.94145188432738));
#34331=CARTESIAN_POINT('Ctrl Pts',(3.3391842955686,1.75000000000001,3.03108891324553));
#34332=CARTESIAN_POINT('Ctrl Pts',(2.84579300863683,3.32679491924311,2.12072594216369));
#34333=CARTESIAN_POINT('',(2.84579300863683,-0.173205080756887,3.94145188432738));
#34334=CARTESIAN_POINT('Ctrl Pts',(2.84579300863683,-0.173205080756887,
3.94145188432738));
#34335=CARTESIAN_POINT('Ctrl Pts',(2.85025803029788,6.97358837342676E-15,
3.94145188432738));
#34336=CARTESIAN_POINT('Ctrl Pts',(2.84579300863683,0.173205080756888,3.94145188432738));
#34337=CARTESIAN_POINT('',(2.84579300863683,-3.32679491924311,2.12072594216369));
#34338=CARTESIAN_POINT('Ctrl Pts',(2.84579300863683,-3.32679491924311,2.12072594216369));
#34339=CARTESIAN_POINT('Ctrl Pts',(3.3391842955686,-1.75,3.03108891324554));
#34340=CARTESIAN_POINT('Ctrl Pts',(2.84579300863683,-0.173205080756886,
3.94145188432738));
#34341=CARTESIAN_POINT('',(2.84579300863683,-3.5,1.82072594216369));
#34342=CARTESIAN_POINT('Ctrl Pts',(2.84579300863683,-3.5,1.82072594216369));
#34343=CARTESIAN_POINT('Ctrl Pts',(2.85025803029788,-3.41339745962155,1.9707259421637));
#34344=CARTESIAN_POINT('Ctrl Pts',(2.84579300863683,-3.32679491924311,2.12072594216369));
#34345=CARTESIAN_POINT('',(3.10724202769303,-3.5,-5.24027883276575E-16));
#34346=CARTESIAN_POINT('Ctrl Pts',(3.10724202769303,-3.5,-6.19429386851577E-16));
#34347=CARTESIAN_POINT('Ctrl Pts',(3.10724202769303,-3.5,0.855919663339608));
#34348=CARTESIAN_POINT('Ctrl Pts',(2.84579300863683,-3.5,1.82072594216369));
#34349=CARTESIAN_POINT('',(3.2,-3.34203030879952,-4.09280672032477E-16));
#34350=CARTESIAN_POINT('',(2.91157561548264,-3.83322594216369,-4.69434788047936E-16));
#34351=CARTESIAN_POINT('Origin',(3.2,0.,0.));
#34352=CARTESIAN_POINT('',(2.84579300863683,-3.5,-1.82072594216369));
#34353=CARTESIAN_POINT('Ctrl Pts',(2.84579300863683,-3.5,-1.82072594216369));
#34354=CARTESIAN_POINT('Ctrl Pts',(3.10724202769303,-3.5,-0.855919663339607));
#34355=CARTESIAN_POINT('Ctrl Pts',(3.10724202769303,-3.5,-6.19429386851577E-16));
#34356=CARTESIAN_POINT('',(2.84579300863683,-3.32679491924311,-2.12072594216369));
#34357=CARTESIAN_POINT('Ctrl Pts',(2.84579300863683,-3.32679491924311,-2.12072594216369));
#34358=CARTESIAN_POINT('Ctrl Pts',(2.85025803029788,-3.41339745962156,-1.97072594216368));
#34359=CARTESIAN_POINT('Ctrl Pts',(2.84579300863683,-3.5,-1.82072594216369));
#34360=CARTESIAN_POINT('',(2.84579300863683,-0.173205080756888,-3.94145188432738));
#34361=CARTESIAN_POINT('Ctrl Pts',(2.84579300863683,-0.173205080756888,
-3.94145188432738));
#34362=CARTESIAN_POINT('Ctrl Pts',(3.3391842955686,-1.75,-3.03108891324553));
#34363=CARTESIAN_POINT('Ctrl Pts',(2.84579300863683,-3.32679491924311,-2.12072594216369));
#34364=CARTESIAN_POINT('',(2.84579300863683,0.173205080756887,-3.94145188432738));
#34365=CARTESIAN_POINT('Ctrl Pts',(2.84579300863683,0.173205080756887,-3.94145188432738));
#34366=CARTESIAN_POINT('Ctrl Pts',(2.85025803029788,-6.80011602582908E-15,
-3.94145188432738));
#34367=CARTESIAN_POINT('Ctrl Pts',(2.84579300863683,-0.173205080756888,
-3.94145188432738));
#34368=CARTESIAN_POINT('',(2.84579300863683,3.32679491924311,-2.12072594216369));
#34369=CARTESIAN_POINT('Ctrl Pts',(2.84579300863683,3.32679491924311,-2.12072594216369));
#34370=CARTESIAN_POINT('Ctrl Pts',(3.3391842955686,1.74999999999999,-3.03108891324554));
#34371=CARTESIAN_POINT('Ctrl Pts',(2.84579300863683,0.173205080756888,-3.94145188432738));
#34372=CARTESIAN_POINT('Ctrl Pts',(2.84579300863683,3.5,-1.82072594216369));
#34373=CARTESIAN_POINT('Ctrl Pts',(2.85025803029788,3.41339745962155,-1.9707259421637));
#34374=CARTESIAN_POINT('Ctrl Pts',(2.84579300863683,3.32679491924311,-2.12072594216369));
#34375=CARTESIAN_POINT('Origin',(0.1,0.,0.));
#34376=CARTESIAN_POINT('',(0.,2.75545529808154E-16,2.25));
#34377=CARTESIAN_POINT('Origin',(0.,0.,0.));
#34378=CARTESIAN_POINT('',(0.2,-2.51052593825207E-16,2.05));
#34379=CARTESIAN_POINT('',(0.1,2.63299061816681E-16,2.15));
#34380=CARTESIAN_POINT('Origin',(0.2,0.,0.));
#34381=CARTESIAN_POINT('Origin',(0.,0.,0.));
#34382=CARTESIAN_POINT('',(3.,2.51052593825207E-16,2.05));
#34383=CARTESIAN_POINT('',(0.,-2.51052593825207E-16,2.05));
#34384=CARTESIAN_POINT('Origin',(3.,0.,0.));
#34385=CARTESIAN_POINT('Origin',(0.,0.,0.));
#34386=CARTESIAN_POINT('',(0.,-3.34203030879952,4.09280672032477E-16));
#34387=CARTESIAN_POINT('Origin',(0.,0.,0.));
#34388=CARTESIAN_POINT('Origin',(3.1,0.,0.));
#34389=CARTESIAN_POINT('',(3.2,-2.75545529808154E-16,2.25));
#34390=CARTESIAN_POINT('Origin',(3.2,0.,0.));
#34391=CARTESIAN_POINT('',(3.1,-2.63299061816681E-16,2.15));
#34392=CARTESIAN_POINT('Origin',(3.2,0.,0.));
#34393=CARTESIAN_POINT('Origin',(0.,4.5102810375397E-16,3.94145188432738));
#34394=CARTESIAN_POINT('',(0.354206991363169,0.173205080756889,3.94145188432738));
#34395=CARTESIAN_POINT('',(0.,0.173205080756888,3.94145188432738));
#34396=CARTESIAN_POINT('',(0.35420699136317,-0.173205080756887,3.94145188432738));
#34397=CARTESIAN_POINT('Ctrl Pts',(0.354206991363169,0.173205080756889,
3.94145188432738));
#34398=CARTESIAN_POINT('Ctrl Pts',(0.349741969702116,-5.62050406216485E-15,
3.94145188432738));
#34399=CARTESIAN_POINT('Ctrl Pts',(0.35420699136317,-0.173205080756887,
3.94145188432738));
#34400=CARTESIAN_POINT('',(0.,-0.173205080756887,3.94145188432738));
#34401=CARTESIAN_POINT('Origin',(0.,2.47467555702478E-16,4.04145188432738));
#34402=CARTESIAN_POINT('',(0.35420699136317,-3.32679491924311,2.12072594216369));
#34403=CARTESIAN_POINT('Ctrl Pts',(0.35420699136317,-0.173205080756887,
3.94145188432738));
#34404=CARTESIAN_POINT('Ctrl Pts',(-0.139184295568602,-1.75,3.03108891324553));
#34405=CARTESIAN_POINT('Ctrl Pts',(0.35420699136317,-3.32679491924311,2.12072594216369));
#34406=CARTESIAN_POINT('',(0.,-3.32679491924311,2.12072594216369));
#34407=CARTESIAN_POINT('Origin',(0.288424384517358,0.,0.));
#34408=CARTESIAN_POINT('',(0.0927579723069723,-3.5,-5.85970821961734E-16));
#34409=CARTESIAN_POINT('',(0.288424384517358,-3.83322594216369,-4.69434788047936E-16));
#34410=CARTESIAN_POINT('',(0.35420699136317,-3.5,1.82072594216369));
#34411=CARTESIAN_POINT('Ctrl Pts',(0.35420699136317,-3.5,1.82072594216369));
#34412=CARTESIAN_POINT('Ctrl Pts',(0.0927579723069726,-3.5,0.855919663339608));
#34413=CARTESIAN_POINT('Ctrl Pts',(0.0927579723069723,-3.5,-7.43315264221894E-16));
#34414=CARTESIAN_POINT('Ctrl Pts',(0.35420699136317,-3.32679491924311,2.12072594216369));
#34415=CARTESIAN_POINT('Ctrl Pts',(0.349741969702116,-3.41339745962156,
1.97072594216368));
#34416=CARTESIAN_POINT('Ctrl Pts',(0.35420699136317,-3.5,1.82072594216369));
#34417=CARTESIAN_POINT('Ctrl Pts',(0.35420699136317,3.32679491924311,2.12072594216369));
#34418=CARTESIAN_POINT('Ctrl Pts',(-0.139184295568602,1.75,3.03108891324554));
#34419=CARTESIAN_POINT('Ctrl Pts',(0.354206991363169,0.173205080756889,
3.94145188432738));
#34420=CARTESIAN_POINT('',(0.35420699136317,3.32679491924311,-2.12072594216369));
#34421=CARTESIAN_POINT('Ctrl Pts',(0.35420699136317,3.32679491924311,-2.12072594216369));
#34422=CARTESIAN_POINT('Ctrl Pts',(0.349741969702117,3.41339745962156,-1.97072594216369));
#34423=CARTESIAN_POINT('Ctrl Pts',(0.35420699136317,3.5,-1.82072594216369));
#34424=CARTESIAN_POINT('',(0.35420699136317,0.173205080756888,-3.94145188432738));
#34425=CARTESIAN_POINT('Ctrl Pts',(0.35420699136317,0.173205080756887,-3.94145188432738));
#34426=CARTESIAN_POINT('Ctrl Pts',(-0.1391842955686,1.75,-3.03108891324553));
#34427=CARTESIAN_POINT('Ctrl Pts',(0.35420699136317,3.32679491924311,-2.12072594216369));
#34428=CARTESIAN_POINT('',(0.35420699136317,-0.173205080756888,-3.94145188432738));
#34429=CARTESIAN_POINT('Ctrl Pts',(0.35420699136317,-0.173205080756888,
-3.94145188432738));
#34430=CARTESIAN_POINT('Ctrl Pts',(0.349741969702117,6.1409211049579E-15,
-3.94145188432738));
#34431=CARTESIAN_POINT('Ctrl Pts',(0.35420699136317,0.173205080756888,-3.94145188432738));
#34432=CARTESIAN_POINT('',(0.35420699136317,-3.32679491924311,-2.12072594216369));
#34433=CARTESIAN_POINT('Ctrl Pts',(0.35420699136317,-3.32679491924311,-2.12072594216369));
#34434=CARTESIAN_POINT('Ctrl Pts',(-0.139184295568601,-1.75,-3.03108891324554));
#34435=CARTESIAN_POINT('Ctrl Pts',(0.35420699136317,-0.173205080756889,
-3.94145188432738));
#34436=CARTESIAN_POINT('',(0.354206991363169,-3.5,-1.82072594216369));
#34437=CARTESIAN_POINT('Ctrl Pts',(0.354206991363169,-3.5,-1.82072594216369));
#34438=CARTESIAN_POINT('Ctrl Pts',(0.349741969702116,-3.41339745962155,
-1.9707259421637));
#34439=CARTESIAN_POINT('Ctrl Pts',(0.35420699136317,-3.32679491924311,-2.12072594216369));
#34440=CARTESIAN_POINT('Ctrl Pts',(0.0927579723069723,-3.5,-7.43315264221894E-16));
#34441=CARTESIAN_POINT('Ctrl Pts',(0.092757972306972,-3.5,-0.85591966333961));
#34442=CARTESIAN_POINT('Ctrl Pts',(0.354206991363169,-3.5,-1.82072594216369));
#34443=CARTESIAN_POINT('Origin',(0.,-3.41339745962156,1.97072594216369));
#34444=CARTESIAN_POINT('',(0.,-3.5,1.82072594216369));
#34445=CARTESIAN_POINT('Origin',(0.,-3.5,2.02072594216369));
#34446=CARTESIAN_POINT('',(0.,-3.5,-1.82072594216369));
#34447=CARTESIAN_POINT('Origin',(0.,-3.41339745962156,-1.97072594216369));
#34448=CARTESIAN_POINT('',(0.,-3.32679491924311,-2.12072594216369));
#34449=CARTESIAN_POINT('Origin',(0.,3.41339745962155,-1.97072594216369));
#34450=CARTESIAN_POINT('',(0.,3.32679491924311,-2.12072594216369));
#34451=CARTESIAN_POINT('Origin',(0.,-7.42402667107435E-16,-4.04145188432738));
#34452=CARTESIAN_POINT('',(0.,0.173205080756887,-3.94145188432738));
#34453=CARTESIAN_POINT('Origin',(0.,-5.20417042793042E-16,-3.94145188432738));
#34454=CARTESIAN_POINT('',(0.,-0.173205080756888,-3.94145188432738));
#34455=CARTESIAN_POINT('Origin',(0.,-3.5,-2.02072594216369));
#34456=CARTESIAN_POINT('Origin',(0.,3.5,2.02072594216369));
#37164=UNCERTAINTY_MEASURE_WITH_UNIT(LENGTH_MEASURE(0.01),#37182,
'DISTANCE_ACCURACY_VALUE',
'Maximum model space distance between geometric entities at asserted c
onnectivities');
#37166=UNCERTAINTY_MEASURE_WITH_UNIT(LENGTH_MEASURE(0.01),#37182,
'DISTANCE_ACCURACY_VALUE',
'Maximum model space distance between geometric entities at asserted c
onnectivities');
#37179=(
GEOMETRIC_REPRESENTATION_CONTEXT(3)
GLOBAL_UNCERTAINTY_ASSIGNED_CONTEXT((#37164))
GLOBAL_UNIT_ASSIGNED_CONTEXT((#37182,#37184,#37185))
REPRESENTATION_CONTEXT('','3D')
);
#37181=(
GEOMETRIC_REPRESENTATION_CONTEXT(3)
GLOBAL_UNCERTAINTY_ASSIGNED_CONTEXT((#37166))
GLOBAL_UNIT_ASSIGNED_CONTEXT((#37182,#37184,#37185))
REPRESENTATION_CONTEXT('','3D')
);
#37182=(
LENGTH_UNIT()
NAMED_UNIT(*)
SI_UNIT(.MILLI.,.METRE.)
);
#37184=(
NAMED_UNIT(*)
PLANE_ANGLE_UNIT()
SI_UNIT($,.RADIAN.)
);
#37185=(
NAMED_UNIT(*)
SI_UNIT($,.STERADIAN.)
SOLID_ANGLE_UNIT()
);
#37198=SHAPE_DEFINITION_REPRESENTATION(#37212,#37249);
#37212=PRODUCT_DEFINITION_SHAPE('',$,#37264);
#37249=SHAPE_REPRESENTATION('',(#16013),#37179);
#37251=PRODUCT_DEFINITION_CONTEXT('part definition',#37295,'design');
#37264=PRODUCT_DEFINITION('2026-10-20-13-24-01-496',
'10_ISO_4032_Nut_M4',#37278,#37251);
#37278=PRODUCT_DEFINITION_FORMATION('',$,#37309);
#37295=APPLICATION_CONTEXT(
'Core Data for Automotive Mechanical Design Process');
#37296=PRODUCT_CONTEXT('part definition',#37295,'mechanical');
#37309=PRODUCT('2026-10-20-13-24-01-496','10_ISO_4032_Nut_M4',$,(#37296));
#37374=COLOUR_RGB('Black',0.12,0.14,0.17);
#37375=FILL_AREA_STYLE_COLOUR('',#37374);
#37376=FILL_AREA_STYLE('',(#37375));
#37377=SURFACE_STYLE_FILL_AREA(#37376);
#37378=SURFACE_SIDE_STYLE('',(#37377));
#37379=SURFACE_STYLE_USAGE(.BOTH.,#37378);
#37380=PRESENTATION_STYLE_ASSIGNMENT((#37379));
ENDSEC;
END-ISO-10303-21;
